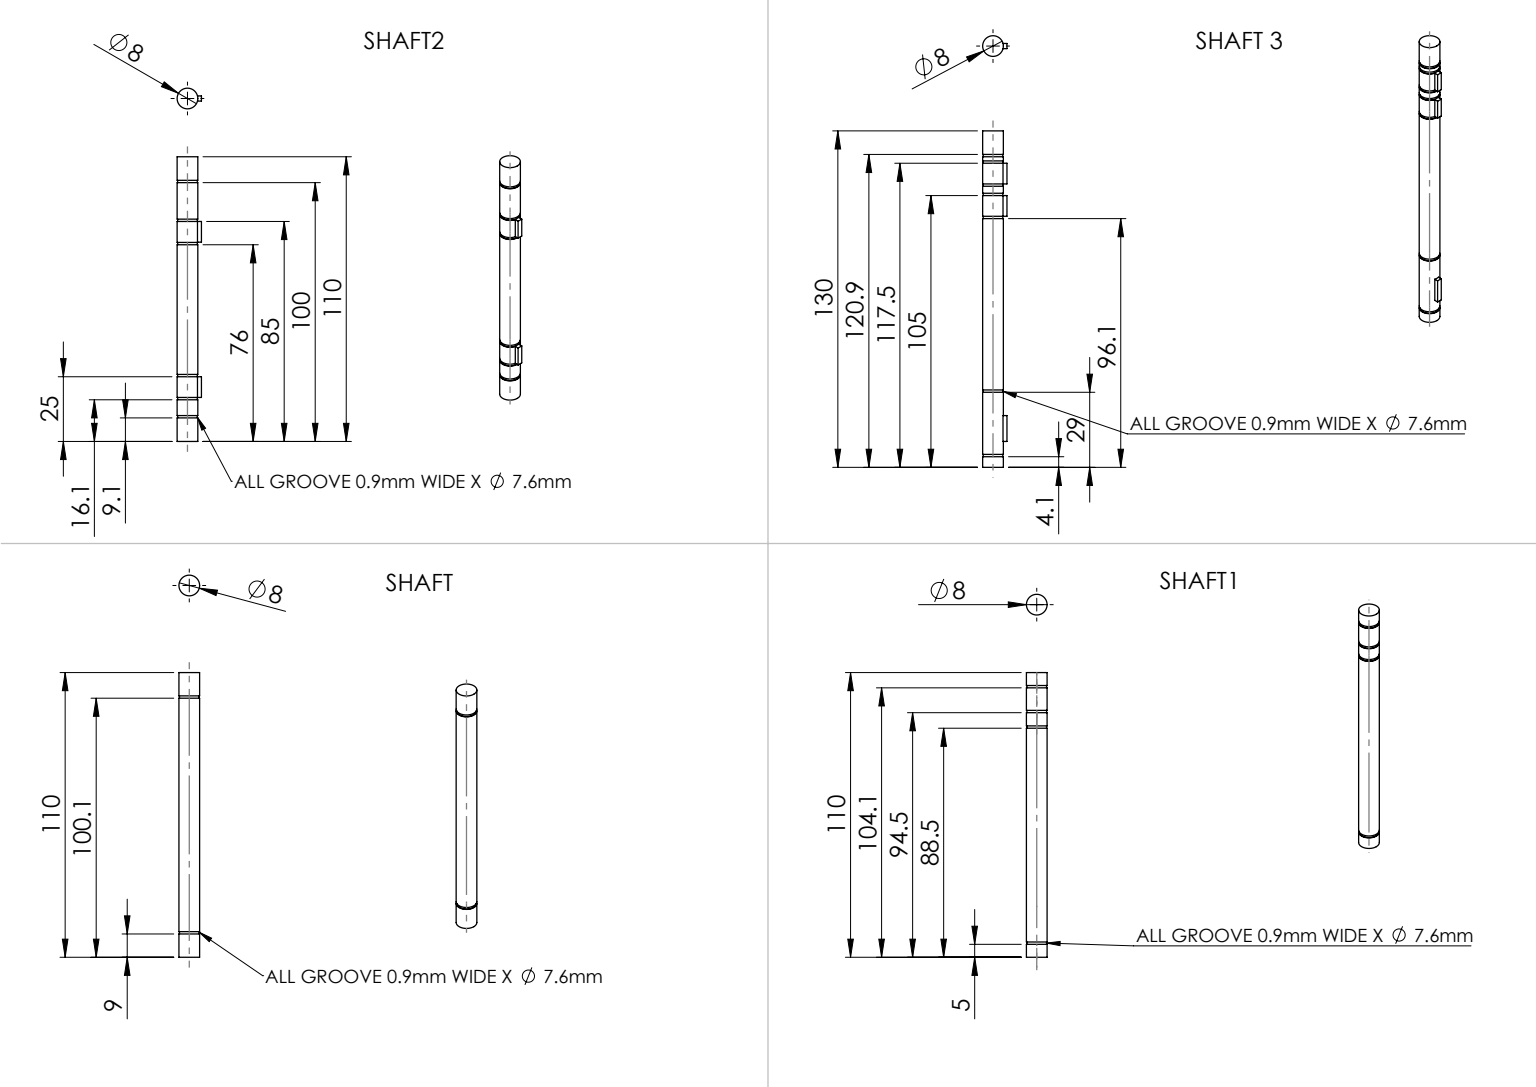
ISO-10303-21;
HEADER;
FILE_DESCRIPTION (('STEP AP214'),
    '1' );
FILE_NAME ('shaft.step',
    '2026-09-28T15:49:00',
    ( '' ),
    ( '' ),
    'SwSTEP 2.0',
    'SolidWorks 2026',
    '' );
FILE_SCHEMA (( 'AUTOMOTIVE_DESIGN' ));
ENDSEC;

DATA;
#80=ADVANCED_FACE ( 'NONE', ( #27547, #5915 ), #12161, .T. ) ;
#129=COLOUR_RGB ( '', 0.40784314, 0.44705882, 0.49803922) ;
#234=AXIS2_PLACEMENT_3D ( 'NONE', #3071, #14027, #25022 ) ;
#259=ADVANCED_FACE ( 'NONE', ( #12521 ), #20953, .T. ) ;
#263=CARTESIAN_POINT ( 'NONE',  ( 0.000000000000000000, -2.710505431213761085E-17, 54.99999999999999289 ) ) ;
#301=ORIENTED_EDGE ( 'NONE', *, *, #5401, .F. ) ;
#489=CARTESIAN_POINT ( 'NONE',  ( 4.000000000000000000, 4.627536653468036720E-16, 45.99999999999998579 ) ) ;
#517=DIRECTION ( 'NONE',  ( -1.000000000000000000, 0.000000000000000000, 0.000000000000000000 ) ) ;
#545=CIRCLE ( 'NONE', #10351, 4.000000000000000000 ) ;
#600=DIRECTION ( 'NONE',  ( -1.000000000000000000, 0.000000000000000000, 0.000000000000000000 ) ) ;
#613=FACE_OUTER_BOUND ( 'NONE', #17801, .T. ) ;
#665=PLANE ( 'NONE',  #1337 ) ;
#705=ADVANCED_FACE ( 'NONE', ( #23823 ), #18225, .T. ) ;
#706=DIRECTION ( 'NONE',  ( 1.000000000000000000, 0.000000000000000000, 0.000000000000000000 ) ) ;
#829=DIRECTION ( 'NONE',  ( 0.000000000000000000, 0.000000000000000000, -1.000000000000000000 ) ) ;
#842=VECTOR ( 'NONE', #18131, 1000.000000000000000 ) ;
#860=DIRECTION ( 'NONE',  ( 1.000000000000000000, 0.000000000000000000, 0.000000000000000000 ) ) ;
#903=CIRCLE ( 'NONE', #21584, 3.799999999999999822 ) ;
#937=SHAPE_REPRESENTATION_RELATIONSHIP ( 'NONE' , 'NONE' ,  #15534, #14621 ) ;
#1059=DIRECTION ( 'NONE',  ( 0.000000000000000000, 0.000000000000000000, -1.000000000000000000 ) ) ;
#1066=DIRECTION ( 'NONE',  ( 0.000000000000000000, 0.000000000000000000, -1.000000000000000000 ) ) ;
#1122=SURFACE_STYLE_USAGE ( .BOTH. , #3832 ) ;
#1124=EDGE_LOOP ( 'NONE', ( #30644, #31350 ) ) ;
#1169=EDGE_CURVE ( 'NONE', #3555, #2086, #8831, .T. ) ;
#1291=( LENGTH_UNIT ( ) NAMED_UNIT ( * ) SI_UNIT ( .MILLI., .METRE. ) );
#1322=CYLINDRICAL_SURFACE ( 'NONE', #32817, 3.799999999999999822 ) ;
#1337=AXIS2_PLACEMENT_3D ( 'NONE', #22806, #33808, #28399 ) ;
#1373=EDGE_LOOP ( 'NONE', ( #13603, #23594 ) ) ;
#1375=AXIS2_PLACEMENT_3D ( 'NONE', #34845, #33025, #24748 ) ;
#1477=DIRECTION ( 'NONE',  ( 0.000000000000000000, 0.000000000000000000, 1.000000000000000000 ) ) ;
#1539=DIRECTION ( 'NONE',  ( 0.000000000000000000, 0.000000000000000000, -1.000000000000000000 ) ) ;
#1577=AXIS2_PLACEMENT_3D ( 'NONE', #7509, #1763, #18490 ) ;
#1686=FACE_OUTER_BOUND ( 'NONE', #17486, .T. ) ;
#1753=EDGE_CURVE ( 'NONE', #16353, #3289, #16331, .T. ) ;
#1763=DIRECTION ( 'NONE',  ( 0.000000000000000000, 0.000000000000000000, -1.000000000000000000 ) ) ;
#1866=CARTESIAN_POINT ( 'NONE',  ( 0.000000000000000000, -2.710505431213761085E-17, 45.10000000000000142 ) ) ;
#1902=FACE_OUTER_BOUND ( 'NONE', #33338, .T. ) ;
#2086=VERTEX_POINT ( 'NONE', #489 ) ;
#2220=FACE_OUTER_BOUND ( 'NONE', #24548, .T. ) ;
#2301=AXIS2_PLACEMENT_3D ( 'NONE', #14881, #3933, #26600 ) ;
#2321=CARTESIAN_POINT ( 'NONE',  ( 0.000000000000000000, -2.710505431213761085E-17, -45.10000000000000142 ) ) ;
#2331=ADVANCED_FACE ( 'NONE', ( #31792 ), #18100, .T. ) ;
#2429=DIRECTION ( 'NONE',  ( 0.000000000000000000, 0.000000000000000000, -1.000000000000000000 ) ) ;
#2463=ORIENTED_EDGE ( 'NONE', *, *, #5481, .F. ) ;
#2522=APPLICATION_CONTEXT ( 'automotive_design' ) ;
#2817=AXIS2_PLACEMENT_3D ( 'NONE', #31798, #6779, #34335 ) ;
#2884=CARTESIAN_POINT ( 'NONE',  ( 0.000000000000000000, -2.710505431213761085E-17, -45.10000000000000142 ) ) ;
#2978=FILL_AREA_STYLE_COLOUR ( '', #129 ) ;
#3001=APPLICATION_CONTEXT ( 'automotive_design' ) ;
#3071=CARTESIAN_POINT ( 'NONE',  ( 0.000000000000000000, -2.710505431213761085E-17, -45.10000000000000142 ) ) ;
#3181=AXIS2_PLACEMENT_3D ( 'NONE', #2884, #32755, #11149 ) ;
#3219=CARTESIAN_POINT ( 'NONE',  ( 0.000000000000000000, -2.710505431213761085E-17, -54.99999999999999289 ) ) ;
#3289=VERTEX_POINT ( 'NONE', #18576 ) ;
#3320=DIRECTION ( 'NONE',  ( -1.000000000000000000, 0.000000000000000000, 0.000000000000000000 ) ) ;
#3382=CARTESIAN_POINT ( 'NONE',  ( 4.000000000000000000, 4.627536653468036720E-16, 45.10000000000000142 ) ) ;
#3555=VERTEX_POINT ( 'NONE', #12061 ) ;
#3639=AXIS2_PLACEMENT_3D ( 'NONE', #10281, #27025, #32239 ) ;
#3651=CARTESIAN_POINT ( 'NONE',  ( -3.799999999999999822, 4.382607293638566128E-16, 45.99999999999998579 ) ) ;
#3674=DIRECTION ( 'NONE',  ( 0.000000000000000000, 0.000000000000000000, -1.000000000000000000 ) ) ;
#3832=SURFACE_SIDE_STYLE ('',( #7220 ) ) ;
#3850=CARTESIAN_POINT ( 'NONE',  ( 0.000000000000000000, -2.710505431213761085E-17, 45.10000000000000142 ) ) ;
#3852=AXIS2_PLACEMENT_3D ( 'NONE', #24445, #10762, #21729 ) ;
#3933=DIRECTION ( 'NONE',  ( 0.000000000000000000, 0.000000000000000000, -1.000000000000000000 ) ) ;
#3969=CIRCLE ( 'NONE', #24668, 4.000000000000000000 ) ;
#4052=ORIENTED_EDGE ( 'NONE', *, *, #12390, .F. ) ;
#4364=FILL_AREA_STYLE_COLOUR ( '', #22512 ) ;
#4391=VECTOR ( 'NONE', #18228, 1000.000000000000000 ) ;
#4412=ORIENTED_EDGE ( 'NONE', *, *, #11688, .F. ) ;
#4594=AXIS2_PLACEMENT_3D ( 'NONE', #2321, #12751, #21197 ) ;
#4692=ADVANCED_FACE ( 'NONE', ( #1902 ), #12877, .T. ) ;
#4738=ORIENTED_EDGE ( 'NONE', *, *, #29385, .T. ) ;
#4795=LINE ( 'NONE', #15738, #14958 ) ;
#4961=AXIS2_PLACEMENT_3D ( 'NONE', #6185, #14096, #3320 ) ;
#4987=ORIENTED_EDGE ( 'NONE', *, *, #32459, .F. ) ;
#5002=AXIS2_PLACEMENT_3D ( 'NONE', #29082, #1539, #9453 ) ;
#5030=CIRCLE ( 'NONE', #26307, 3.799999999999999822 ) ;
#5259=ORIENTED_EDGE ( 'NONE', *, *, #9211, .F. ) ;
#5302=VECTOR ( 'NONE', #5780, 1000.000000000000000 ) ;
#5401=EDGE_CURVE ( 'NONE', #13238, #3289, #31820, .T. ) ;
#5481=EDGE_CURVE ( 'NONE', #19767, #30356, #11769, .T. ) ;
#5780=DIRECTION ( 'NONE',  ( 0.000000000000000000, 0.000000000000000000, -1.000000000000000000 ) ) ;
#5847=DIRECTION ( 'NONE',  ( -1.000000000000000000, 0.000000000000000000, 0.000000000000000000 ) ) ;
#5885=MECHANICAL_DESIGN_GEOMETRIC_PRESENTATION_REPRESENTATION('',(#8745),#32334);
#5915=FACE_OUTER_BOUND ( 'NONE', #1124, .T. ) ;
#6079=FACE_OUTER_BOUND ( 'NONE', #30683, .T. ) ;
#6185=CARTESIAN_POINT ( 'NONE',  ( 0.000000000000000000, -2.710505431213761085E-17, 45.10000000000000142 ) ) ;
#6239=EDGE_CURVE ( 'NONE', #13527, #8697, #34844, .T. ) ;
#6412=ORIENTED_EDGE ( 'NONE', *, *, #25778, .T. ) ;
#6415=CARTESIAN_POINT ( 'NONE',  ( 0.000000000000000000, -2.710505431213761085E-17, -45.10000000000000142 ) ) ;
#6460=CIRCLE ( 'NONE', #26601, 4.000000000000000000 ) ;
#6648=EDGE_CURVE ( 'NONE', #7361, #16353, #29410, .T. ) ;
#6779=DIRECTION ( 'NONE',  ( 0.000000000000000000, 0.000000000000000000, -1.000000000000000000 ) ) ;
#6807=CARTESIAN_POINT ( 'NONE',  ( 0.000000000000000000, -2.710505431213761085E-17, 45.99999999999998579 ) ) ;
#6995=MECHANICAL_DESIGN_GEOMETRIC_PRESENTATION_REPRESENTATION('',(#32297),#16755);
#7085=EDGE_CURVE ( 'NONE', #7361, #13238, #14160, .T. ) ;
#7154=CIRCLE ( 'NONE', #28440, 4.000000000000000000 ) ;
#7168=ORIENTED_EDGE ( 'NONE', *, *, #6239, .T. ) ;
#7220=SURFACE_STYLE_FILL_AREA ( #12453 ) ;
#7250=DIRECTION ( 'NONE',  ( 1.000000000000000000, 0.000000000000000000, 0.000000000000000000 ) ) ;
#7361=VERTEX_POINT ( 'NONE', #3382 ) ;
#7463=PRODUCT_DEFINITION_FORMATION_WITH_SPECIFIED_SOURCE ( 'ANY', '', #15545, .NOT_KNOWN. ) ;
#7509=CARTESIAN_POINT ( 'NONE',  ( 0.000000000000000000, -2.710505431213761085E-17, 45.99999999999998579 ) ) ;
#7548=DIRECTION ( 'NONE',  ( 0.000000000000000000, 0.000000000000000000, -1.000000000000000000 ) ) ;
#7803=AXIS2_PLACEMENT_3D ( 'NONE', #26250, #12925, #18316 ) ;
#7814=PRESENTATION_STYLE_ASSIGNMENT (( #10893 ) ) ;
#7886=CIRCLE ( 'NONE', #1577, 3.799999999999999822 ) ;
#7908=ORIENTED_EDGE ( 'NONE', *, *, #10208, .F. ) ;
#7979=ORIENTED_EDGE ( 'NONE', *, *, #9211, .T. ) ;
#8005=DIRECTION ( 'NONE',  ( 1.000000000000000000, 0.000000000000000000, 0.000000000000000000 ) ) ;
#8074=LINE ( 'NONE', #35463, #29789 ) ;
#8214=CARTESIAN_POINT ( 'NONE',  ( 0.000000000000000000, -2.710505431213761085E-17, 45.99999999999998579 ) ) ;
#8262=CARTESIAN_POINT ( 'NONE',  ( -3.799999999999999822, 4.382607293638566128E-16, 45.10000000000000142 ) ) ;
#8503=CARTESIAN_POINT ( 'NONE',  ( 0.000000000000000000, -2.710505431213761085E-17, 45.10000000000000142 ) ) ;
#8510=FACE_OUTER_BOUND ( 'NONE', #22264, .T. ) ;
#8538=DIRECTION ( 'NONE',  ( 0.000000000000000000, 0.000000000000000000, -1.000000000000000000 ) ) ;
#8581=ORIENTED_EDGE ( 'NONE', *, *, #5481, .T. ) ;
#8669=DIRECTION ( 'NONE',  ( -1.000000000000000000, 0.000000000000000000, 0.000000000000000000 ) ) ;
#8697=VERTEX_POINT ( 'NONE', #28414 ) ;
#8745=STYLED_ITEM ( 'NONE', ( #7814 ), #22652 ) ;
#8826=ORIENTED_EDGE ( 'NONE', *, *, #5401, .T. ) ;
#8827=PRODUCT_DEFINITION ( 'UNKNOWN', '', #7463, #25263 ) ;
#8831=LINE ( 'NONE', #23595, #14532 ) ;
#8949=LINE ( 'NONE', #17051, #16731 ) ;
#8986=ORIENTED_EDGE ( 'NONE', *, *, #10627, .F. ) ;
#9049=EDGE_CURVE ( 'NONE', #15222, #24982, #7886, .T. ) ;
#9170=EDGE_LOOP ( 'NONE', ( #9922, #6412, #7168, #12046 ) ) ;
#9211=EDGE_CURVE ( 'NONE', #24982, #15222, #5030, .T. ) ;
#9344=CIRCLE ( 'NONE', #17965, 3.799999999999999822 ) ;
#9453=DIRECTION ( 'NONE',  ( -1.000000000000000000, 0.000000000000000000, 0.000000000000000000 ) ) ;
#9506=CARTESIAN_POINT ( 'NONE',  ( -4.000000000000000000, -2.710505431213761085E-17, 54.99999999999999289 ) ) ;
#9622=ADVANCED_FACE ( 'NONE', ( #16968 ), #11414, .T. ) ;
#9922=ORIENTED_EDGE ( 'NONE', *, *, #12376, .T. ) ;
#10022=CIRCLE ( 'NONE', #14602, 3.799999999999999822 ) ;
#10134=DIRECTION ( 'NONE',  ( 0.000000000000000000, 0.000000000000000000, 1.000000000000000000 ) ) ;
#10208=EDGE_CURVE ( 'NONE', #3289, #16353, #24161, .T. ) ;
#10281=CARTESIAN_POINT ( 'NONE',  ( 0.000000000000000000, -2.710505431213761085E-17, 54.99999999999999289 ) ) ;
#10322=CARTESIAN_POINT ( 'NONE',  ( 0.000000000000000000, -2.710505431213761085E-17, 45.10000000000000142 ) ) ;
#10341=DIRECTION ( 'NONE',  ( 1.000000000000000000, 0.000000000000000000, 0.000000000000000000 ) ) ;
#10351=AXIS2_PLACEMENT_3D ( 'NONE', #3219, #14181, #19568 ) ;
#10491=ORIENTED_EDGE ( 'NONE', *, *, #25778, .F. ) ;
#10575=DIRECTION ( 'NONE',  ( 0.000000000000000000, 0.000000000000000000, -1.000000000000000000 ) ) ;
#10627=EDGE_CURVE ( 'NONE', #19767, #20378, #4795, .T. ) ;
#10693=DIRECTION ( 'NONE',  ( 0.000000000000000000, 0.000000000000000000, 1.000000000000000000 ) ) ;
#10762=DIRECTION ( 'NONE',  ( 0.000000000000000000, 0.000000000000000000, -1.000000000000000000 ) ) ;
#10825=CARTESIAN_POINT ( 'NONE',  ( 3.799999999999999822, -2.710505431213761085E-17, 45.10000000000000142 ) ) ;
#10893=SURFACE_STYLE_USAGE ( .BOTH. , #13583 ) ;
#11077=AXIS2_PLACEMENT_3D ( 'NONE', #16118, #32342, #27136 ) ;
#11099=ADVANCED_FACE ( 'NONE', ( #1686 ), #1322, .T. ) ;
#11149=DIRECTION ( 'NONE',  ( -1.000000000000000000, 0.000000000000000000, 0.000000000000000000 ) ) ;
#11171=CARTESIAN_POINT ( 'NONE',  ( 0.000000000000000000, -2.710505431213761085E-17, 54.99999999999999289 ) ) ;
#11189=ORIENTED_EDGE ( 'NONE', *, *, #25405, .F. ) ;
#11218=CARTESIAN_POINT ( 'NONE',  ( -3.799999999999999822, 4.382607293638566128E-16, 45.10000000000000142 ) ) ;
#11243=CARTESIAN_POINT ( 'NONE',  ( 0.000000000000000000, -2.710505431213761085E-17, -46.00000000000000000 ) ) ;
#11353=FACE_OUTER_BOUND ( 'NONE', #1373, .T. ) ;
#11414=CYLINDRICAL_SURFACE ( 'NONE', #29782, 4.000000000000000000 ) ;
#11521=PLANE ( 'NONE',  #18467 ) ;
#11646=FACE_BOUND ( 'NONE', #33527, .T. ) ;
#11688=EDGE_CURVE ( 'NONE', #30356, #28584, #8949, .T. ) ;
#11734=PLANE ( 'NONE',  #16422 ) ;
#11769=CIRCLE ( 'NONE', #12943, 3.799999999999999822 ) ;
#11877=ADVANCED_FACE ( 'NONE', ( #2220 ), #26871, .F. ) ;
#11899=VERTEX_POINT ( 'NONE', #13188 ) ;
#12029=CARTESIAN_POINT ( 'NONE',  ( 0.000000000000000000, -2.710505431213761085E-17, 54.99999999999999289 ) ) ;
#12030=DIRECTION ( 'NONE',  ( -1.000000000000000000, 0.000000000000000000, 0.000000000000000000 ) ) ;
#12046=ORIENTED_EDGE ( 'NONE', *, *, #18914, .F. ) ;
#12061=CARTESIAN_POINT ( 'NONE',  ( 4.000000000000000000, 4.627536653468036720E-16, 54.99999999999999289 ) ) ;
#12074=ORIENTED_EDGE ( 'NONE', *, *, #12143, .T. ) ;
#12094=PRESENTATION_STYLE_ASSIGNMENT (( #1122 ) ) ;
#12143=EDGE_CURVE ( 'NONE', #19005, #17954, #21792, .T. ) ;
#12161=PLANE ( 'NONE',  #3181 ) ;
#12211=DIRECTION ( 'NONE',  ( 0.000000000000000000, 0.000000000000000000, 1.000000000000000000 ) ) ;
#12292=DIRECTION ( 'NONE',  ( 0.000000000000000000, 0.000000000000000000, -1.000000000000000000 ) ) ;
#12358=CARTESIAN_POINT ( 'NONE',  ( 4.000000000000000000, 4.627536653468036720E-16, -46.00000000000000000 ) ) ;
#12376=EDGE_CURVE ( 'NONE', #11899, #35547, #28881, .T. ) ;
#12384=DIRECTION ( 'NONE',  ( 0.000000000000000000, 0.000000000000000000, -1.000000000000000000 ) ) ;
#12390=EDGE_CURVE ( 'NONE', #35547, #11899, #6460, .T. ) ;
#12453=FILL_AREA_STYLE ('',( #4364 ) ) ;
#12521=FACE_OUTER_BOUND ( 'NONE', #24417, .T. ) ;
#12557=ORIENTED_EDGE ( 'NONE', *, *, #32459, .T. ) ;
#12625=ORIENTED_EDGE ( 'NONE', *, *, #17612, .F. ) ;
#12725=DIRECTION ( 'NONE',  ( 0.000000000000000000, 0.000000000000000000, 1.000000000000000000 ) ) ;
#12751=DIRECTION ( 'NONE',  ( 0.000000000000000000, 0.000000000000000000, -1.000000000000000000 ) ) ;
#12877=CYLINDRICAL_SURFACE ( 'NONE', #1375, 4.000000000000000000 ) ;
#12925=DIRECTION ( 'NONE',  ( 0.000000000000000000, 0.000000000000000000, -1.000000000000000000 ) ) ;
#12943=AXIS2_PLACEMENT_3D ( 'NONE', #28601, #12384, #12030 ) ;
#13188=CARTESIAN_POINT ( 'NONE',  ( -4.000000000000000000, -2.710505431213761085E-17, -46.00000000000000000 ) ) ;
#13238=VERTEX_POINT ( 'NONE', #19194 ) ;
#13353=ORIENTED_EDGE ( 'NONE', *, *, #12376, .F. ) ;
#13527=VERTEX_POINT ( 'NONE', #32138 ) ;
#13583=SURFACE_SIDE_STYLE ('',( #35568 ) ) ;
#13603=ORIENTED_EDGE ( 'NONE', *, *, #16808, .T. ) ;
#13631=CARTESIAN_POINT ( 'NONE',  ( -3.799999999999999822, -2.710505431213761085E-17, -46.00000000000000000 ) ) ;
#13644=UNCERTAINTY_MEASURE_WITH_UNIT (LENGTH_MEASURE( 1.000000000000000082E-05 ), #23439, 'distance_accuracy_value', 'NONE');
#13913=FACE_BOUND ( 'NONE', #34994, .T. ) ;
#13947=FACE_OUTER_BOUND ( 'NONE', #31979, .T. ) ;
#14027=DIRECTION ( 'NONE',  ( 0.000000000000000000, 0.000000000000000000, -1.000000000000000000 ) ) ;
#14096=DIRECTION ( 'NONE',  ( 0.000000000000000000, 0.000000000000000000, -1.000000000000000000 ) ) ;
#14160=CIRCLE ( 'NONE', #3852, 4.000000000000000000 ) ;
#14163=ORIENTED_EDGE ( 'NONE', *, *, #25405, .T. ) ;
#14177=ORIENTED_EDGE ( 'NONE', *, *, #15082, .F. ) ;
#14181=DIRECTION ( 'NONE',  ( 0.000000000000000000, 0.000000000000000000, 1.000000000000000000 ) ) ;
#14198=LINE ( 'NONE', #8262, #17569 ) ;
#14203=VERTEX_POINT ( 'NONE', #15387 ) ;
#14428=DIRECTION ( 'NONE',  ( 0.000000000000000000, 0.000000000000000000, -1.000000000000000000 ) ) ;
#14459=DIRECTION ( 'NONE',  ( -1.000000000000000000, 0.000000000000000000, 0.000000000000000000 ) ) ;
#14492=ORIENTED_EDGE ( 'NONE', *, *, #10627, .T. ) ;
#14532=VECTOR ( 'NONE', #28823, 1000.000000000000000 ) ;
#14602=AXIS2_PLACEMENT_3D ( 'NONE', #28502, #12292, #31730 ) ;
#14621=ADVANCED_BREP_SHAPE_REPRESENTATION ( '', ( #22652, #21307 ), #24262 ) ;
#14690=CIRCLE ( 'NONE', #4961, 4.000000000000000000 ) ;
#14734=VECTOR ( 'NONE', #10575, 1000.000000000000000 ) ;
#14881=CARTESIAN_POINT ( 'NONE',  ( 0.000000000000000000, -2.710505431213761085E-17, 45.99999999999998579 ) ) ;
#14898=CIRCLE ( 'NONE', #2301, 4.000000000000000000 ) ;
#14913=ORIENTED_EDGE ( 'NONE', *, *, #6648, .T. ) ;
#14958=VECTOR ( 'NONE', #31961, 1000.000000000000000 ) ;
#15082=EDGE_CURVE ( 'NONE', #16940, #14203, #22822, .T. ) ;
#15210=ORIENTED_EDGE ( 'NONE', *, *, #12390, .T. ) ;
#15222=VERTEX_POINT ( 'NONE', #3651 ) ;
#15387=CARTESIAN_POINT ( 'NONE',  ( 3.799999999999999822, -2.710505431213761085E-17, 45.10000000000000142 ) ) ;
#15507=DIRECTION ( 'NONE',  ( -1.000000000000000000, 0.000000000000000000, 0.000000000000000000 ) ) ;
#15534=SHAPE_REPRESENTATION ( 'shaft', ( #21307 ), #24262 ) ;
#15545=PRODUCT ( 'shaft', 'shaft', '', ( #28755 ) ) ;
#15568=ORIENTED_EDGE ( 'NONE', *, *, #21852, .F. ) ;
#15715=ORIENTED_EDGE ( 'NONE', *, *, #7085, .F. ) ;
#15738=CARTESIAN_POINT ( 'NONE',  ( 3.799999999999999822, 4.382607293638566128E-16, -45.10000000000000142 ) ) ;
#16118=CARTESIAN_POINT ( 'NONE',  ( 0.000000000000000000, -2.710505431213761085E-17, -46.00000000000000000 ) ) ;
#16258=FILL_AREA_STYLE ('',( #2978 ) ) ;
#16263=CARTESIAN_POINT ( 'NONE',  ( 0.000000000000000000, -2.710505431213761085E-17, -54.99999999999999289 ) ) ;
#16331=CIRCLE ( 'NONE', #234, 4.000000000000000000 ) ;
#16353=VERTEX_POINT ( 'NONE', #25261 ) ;
#16379=CARTESIAN_POINT ( 'NONE',  ( -4.000000000000000000, -2.710505431213761085E-17, 54.99999999999999289 ) ) ;
#16408=DIRECTION ( 'NONE',  ( 0.000000000000000000, 0.000000000000000000, -1.000000000000000000 ) ) ;
#16422=AXIS2_PLACEMENT_3D ( 'NONE', #22706, #14428, #27620 ) ;
#16631=DIRECTION ( 'NONE',  ( 0.000000000000000000, 0.000000000000000000, 1.000000000000000000 ) ) ;
#16731=VECTOR ( 'NONE', #25717, 1000.000000000000000 ) ;
#16755=( GEOMETRIC_REPRESENTATION_CONTEXT ( 3 ) GLOBAL_UNCERTAINTY_ASSIGNED_CONTEXT ( ( #13644 ) ) GLOBAL_UNIT_ASSIGNED_CONTEXT ( ( #23439, #20712, #29015 ) ) REPRESENTATION_CONTEXT ( 'NONE', 'WORKASPACE' ) );
#16759=ORIENTED_EDGE ( 'NONE', *, *, #1169, .F. ) ;
#16808=EDGE_CURVE ( 'NONE', #19005, #3555, #3969, .T. ) ;
#16838=DIRECTION ( 'NONE',  ( 0.000000000000000000, 0.000000000000000000, -1.000000000000000000 ) ) ;
#16852=UNCERTAINTY_MEASURE_WITH_UNIT (LENGTH_MEASURE( 1.000000000000000082E-05 ), #1291, 'distance_accuracy_value', 'NONE');
#16920=AXIS2_PLACEMENT_3D ( 'NONE', #6415, #829, #29102 ) ;
#16940=VERTEX_POINT ( 'NONE', #11218 ) ;
#16968=FACE_OUTER_BOUND ( 'NONE', #30734, .T. ) ;
#17051=CARTESIAN_POINT ( 'NONE',  ( -3.799999999999999822, -2.710505431213761085E-17, -45.10000000000000142 ) ) ;
#17062=CARTESIAN_POINT ( 'NONE',  ( 0.000000000000000000, -2.710505431213761085E-17, 54.99999999999999289 ) ) ;
#17486=EDGE_LOOP ( 'NONE', ( #14177, #24005, #19107, #22794 ) ) ;
#17569=VECTOR ( 'NONE', #33120, 1000.000000000000000 ) ;
#17612=EDGE_CURVE ( 'NONE', #8697, #13527, #545, .T. ) ;
#17801=EDGE_LOOP ( 'NONE', ( #16759, #19908, #12074, #30354 ) ) ;
#17954=VERTEX_POINT ( 'NONE', #29653 ) ;
#17965=AXIS2_PLACEMENT_3D ( 'NONE', #22666, #2429, #21842 ) ;
#17971=ORIENTED_EDGE ( 'NONE', *, *, #15082, .T. ) ;
#18100=CYLINDRICAL_SURFACE ( 'NONE', #16920, 3.799999999999999822 ) ;
#18131=DIRECTION ( 'NONE',  ( 0.000000000000000000, 0.000000000000000000, -1.000000000000000000 ) ) ;
#18225=CYLINDRICAL_SURFACE ( 'NONE', #25462, 3.799999999999999822 ) ;
#18228=DIRECTION ( 'NONE',  ( 0.000000000000000000, 0.000000000000000000, -1.000000000000000000 ) ) ;
#18292=DIRECTION ( 'NONE',  ( 1.000000000000000000, 0.000000000000000000, 0.000000000000000000 ) ) ;
#18316=DIRECTION ( 'NONE',  ( -1.000000000000000000, 0.000000000000000000, 0.000000000000000000 ) ) ;
#18440=PRODUCT_DEFINITION_SHAPE ( 'NONE', 'NONE',  #8827 ) ;
#18467=AXIS2_PLACEMENT_3D ( 'NONE', #11171, #19951, #706 ) ;
#18490=DIRECTION ( 'NONE',  ( -1.000000000000000000, 0.000000000000000000, 0.000000000000000000 ) ) ;
#18576=CARTESIAN_POINT ( 'NONE',  ( -4.000000000000000000, -2.710505431213761085E-17, -45.10000000000000142 ) ) ;
#18914=EDGE_CURVE ( 'NONE', #11899, #8697, #8074, .T. ) ;
#19005=VERTEX_POINT ( 'NONE', #29470 ) ;
#19041=ADVANCED_FACE ( 'NONE', ( #34877 ), #26593, .T. ) ;
#19107=ORIENTED_EDGE ( 'NONE', *, *, #9049, .T. ) ;
#19128=CARTESIAN_POINT ( 'NONE',  ( -3.799999999999999822, -2.710505431213761085E-17, -45.10000000000000142 ) ) ;
#19194=CARTESIAN_POINT ( 'NONE',  ( -4.000000000000000000, -2.710505431213761085E-17, 45.10000000000000142 ) ) ;
#19323=( NAMED_UNIT ( * ) SI_UNIT ( $, .STERADIAN. ) SOLID_ANGLE_UNIT ( ) );
#19393=ORIENTED_EDGE ( 'NONE', *, *, #12143, .F. ) ;
#19514=DIRECTION ( 'NONE',  ( 0.000000000000000000, 0.000000000000000000, -1.000000000000000000 ) ) ;
#19558=EDGE_CURVE ( 'NONE', #2086, #17954, #14898, .T. ) ;
#19568=DIRECTION ( 'NONE',  ( 1.000000000000000000, 0.000000000000000000, 0.000000000000000000 ) ) ;
#19767=VERTEX_POINT ( 'NONE', #29652 ) ;
#19844=AXIS2_PLACEMENT_3D ( 'NONE', #16263, #16631, #8005 ) ;
#19908=ORIENTED_EDGE ( 'NONE', *, *, #16808, .F. ) ;
#19911=ORIENTED_EDGE ( 'NONE', *, *, #24261, .F. ) ;
#19951=DIRECTION ( 'NONE',  ( 0.000000000000000000, 0.000000000000000000, 1.000000000000000000 ) ) ;
#20293=DIRECTION ( 'NONE',  ( -1.000000000000000000, 0.000000000000000000, 0.000000000000000000 ) ) ;
#20378=VERTEX_POINT ( 'NONE', #22368 ) ;
#20712=( NAMED_UNIT ( * ) PLANE_ANGLE_UNIT ( ) SI_UNIT ( $, .RADIAN. ) );
#20782=AXIS2_PLACEMENT_3D ( 'NONE', #34613, #1477, #29022 ) ;
#20953=CYLINDRICAL_SURFACE ( 'NONE', #5002, 3.799999999999999822 ) ;
#21026=CIRCLE ( 'NONE', #35423, 4.000000000000000000 ) ;
#21197=DIRECTION ( 'NONE',  ( -1.000000000000000000, 0.000000000000000000, 0.000000000000000000 ) ) ;
#21307=AXIS2_PLACEMENT_3D ( 'NONE', #26589, #12725, #18292 ) ;
#21418=FACE_OUTER_BOUND ( 'NONE', #32308, .T. ) ;
#21474=CARTESIAN_POINT ( 'NONE',  ( 0.000000000000000000, -2.710505431213761085E-17, 54.99999999999999289 ) ) ;
#21584=AXIS2_PLACEMENT_3D ( 'NONE', #3850, #31729, #15507 ) ;
#21585=CYLINDRICAL_SURFACE ( 'NONE', #3639, 4.000000000000000000 ) ;
#21599=EDGE_CURVE ( 'NONE', #13238, #7361, #14690, .T. ) ;
#21729=DIRECTION ( 'NONE',  ( -1.000000000000000000, 0.000000000000000000, 0.000000000000000000 ) ) ;
#21792=LINE ( 'NONE', #16379, #5302 ) ;
#21842=DIRECTION ( 'NONE',  ( -1.000000000000000000, 0.000000000000000000, 0.000000000000000000 ) ) ;
#21852=EDGE_CURVE ( 'NONE', #14203, #16940, #903, .T. ) ;
#22075=DIRECTION ( 'NONE',  ( -1.000000000000000000, 0.000000000000000000, 0.000000000000000000 ) ) ;
#22218=ORIENTED_EDGE ( 'NONE', *, *, #9049, .F. ) ;
#22264=EDGE_LOOP ( 'NONE', ( #31167, #15715 ) ) ;
#22368=CARTESIAN_POINT ( 'NONE',  ( 3.799999999999999822, 4.382607293638566128E-16, -46.00000000000000000 ) ) ;
#22512=COLOUR_RGB ( '', 0.40784314, 0.44705882, 0.49803922) ;
#22652=MANIFOLD_SOLID_BREP ( 'Mirror1', #29050 ) ;
#22666=CARTESIAN_POINT ( 'NONE',  ( 0.000000000000000000, -2.710505431213761085E-17, -46.00000000000000000 ) ) ;
#22706=CARTESIAN_POINT ( 'NONE',  ( 0.000000000000000000, -2.710505431213761085E-17, 45.10000000000000142 ) ) ;
#22794=ORIENTED_EDGE ( 'NONE', *, *, #29385, .F. ) ;
#22806=CARTESIAN_POINT ( 'NONE',  ( 0.000000000000000000, -2.710505431213761085E-17, 45.99999999999998579 ) ) ;
#22822=CIRCLE ( 'NONE', #35503, 3.799999999999999822 ) ;
#22924=ORIENTED_EDGE ( 'NONE', *, *, #17612, .T. ) ;
#23248=( NAMED_UNIT ( * ) SI_UNIT ( $, .STERADIAN. ) SOLID_ANGLE_UNIT ( ) );
#23439=( LENGTH_UNIT ( ) NAMED_UNIT ( * ) SI_UNIT ( .MILLI., .METRE. ) );
#23594=ORIENTED_EDGE ( 'NONE', *, *, #25273, .T. ) ;
#23595=CARTESIAN_POINT ( 'NONE',  ( 4.000000000000000000, 4.627536653468036720E-16, 54.99999999999999289 ) ) ;
#23620=( NAMED_UNIT ( * ) PLANE_ANGLE_UNIT ( ) SI_UNIT ( $, .RADIAN. ) );
#23646=EDGE_LOOP ( 'NONE', ( #32024, #14913, #7908, #301 ) ) ;
#23727=ADVANCED_FACE ( 'NONE', ( #6079, #11646 ), #665, .T. ) ;
#23793=LINE ( 'NONE', #10825, #26318 ) ;
#23823=FACE_OUTER_BOUND ( 'NONE', #34061, .T. ) ;
#23934=AXIS2_PLACEMENT_3D ( 'NONE', #17062, #1059, #517 ) ;
#24005=ORIENTED_EDGE ( 'NONE', *, *, #28040, .T. ) ;
#24161=CIRCLE ( 'NONE', #4594, 4.000000000000000000 ) ;
#24252=CARTESIAN_POINT ( 'NONE',  ( 0.000000000000000000, -2.710505431213761085E-17, -46.00000000000000000 ) ) ;
#24261=EDGE_CURVE ( 'NONE', #30356, #19767, #10022, .T. ) ;
#24262=( GEOMETRIC_REPRESENTATION_CONTEXT ( 3 ) GLOBAL_UNCERTAINTY_ASSIGNED_CONTEXT ( ( #16852 ) ) GLOBAL_UNIT_ASSIGNED_CONTEXT ( ( #1291, #23620, #23248 ) ) REPRESENTATION_CONTEXT ( 'NONE', 'WORKASPACE' ) );
#24267=LINE ( 'NONE', #35254, #14734 ) ;
#24417=EDGE_LOOP ( 'NONE', ( #30820, #14492, #4987, #4412 ) ) ;
#24445=CARTESIAN_POINT ( 'NONE',  ( 0.000000000000000000, -2.710505431213761085E-17, 45.10000000000000142 ) ) ;
#24548=EDGE_LOOP ( 'NONE', ( #12625, #35137 ) ) ;
#24668=AXIS2_PLACEMENT_3D ( 'NONE', #21474, #10693, #10341 ) ;
#24748=DIRECTION ( 'NONE',  ( -1.000000000000000000, 0.000000000000000000, 0.000000000000000000 ) ) ;
#24852=ORIENTED_EDGE ( 'NONE', *, *, #18914, .T. ) ;
#24935=PLANE ( 'NONE',  #27924 ) ;
#24982=VERTEX_POINT ( 'NONE', #29710 ) ;
#25022=DIRECTION ( 'NONE',  ( -1.000000000000000000, 0.000000000000000000, 0.000000000000000000 ) ) ;
#25113=CYLINDRICAL_SURFACE ( 'NONE', #30337, 4.000000000000000000 ) ;
#25261=CARTESIAN_POINT ( 'NONE',  ( 4.000000000000000000, 4.627536653468036720E-16, -45.10000000000000142 ) ) ;
#25263=PRODUCT_DEFINITION_CONTEXT ( 'detailed design', #3001, 'design' ) ;
#25273=EDGE_CURVE ( 'NONE', #3555, #19005, #21026, .T. ) ;
#25335=ADVANCED_FACE ( 'NONE', ( #30938 ), #28600, .T. ) ;
#25405=EDGE_CURVE ( 'NONE', #20378, #28584, #27932, .T. ) ;
#25462=AXIS2_PLACEMENT_3D ( 'NONE', #1866, #34807, #34266 ) ;
#25574=ORIENTED_EDGE ( 'NONE', *, *, #25273, .F. ) ;
#25717=DIRECTION ( 'NONE',  ( 0.000000000000000000, 0.000000000000000000, -1.000000000000000000 ) ) ;
#25778=EDGE_CURVE ( 'NONE', #35547, #13527, #24267, .T. ) ;
#26250=CARTESIAN_POINT ( 'NONE',  ( 0.000000000000000000, -2.710505431213761085E-17, -46.00000000000000000 ) ) ;
#26307=AXIS2_PLACEMENT_3D ( 'NONE', #8214, #16838, #22075 ) ;
#26318=VECTOR ( 'NONE', #34776, 1000.000000000000000 ) ;
#26481=ADVANCED_FACE ( 'NONE', ( #21418 ), #21585, .T. ) ;
#26589=CARTESIAN_POINT ( 'NONE',  ( 0.000000000000000000, 0.000000000000000000, 0.000000000000000000 ) ) ;
#26593=CYLINDRICAL_SURFACE ( 'NONE', #2817, 4.000000000000000000 ) ;
#26600=DIRECTION ( 'NONE',  ( -1.000000000000000000, 0.000000000000000000, 0.000000000000000000 ) ) ;
#26601=AXIS2_PLACEMENT_3D ( 'NONE', #24252, #35239, #30012 ) ;
#26861=EDGE_CURVE ( 'NONE', #17954, #2086, #7154, .T. ) ;
#26871=PLANE ( 'NONE',  #20782 ) ;
#26933=( NAMED_UNIT ( * ) PLANE_ANGLE_UNIT ( ) SI_UNIT ( $, .RADIAN. ) );
#27025=DIRECTION ( 'NONE',  ( 0.000000000000000000, 0.000000000000000000, -1.000000000000000000 ) ) ;
#27102=( LENGTH_UNIT ( ) NAMED_UNIT ( * ) SI_UNIT ( .MILLI., .METRE. ) );
#27136=DIRECTION ( 'NONE',  ( -1.000000000000000000, 0.000000000000000000, 0.000000000000000000 ) ) ;
#27547=FACE_BOUND ( 'NONE', #31844, .T. ) ;
#27559=ORIENTED_EDGE ( 'NONE', *, *, #21852, .T. ) ;
#27620=DIRECTION ( 'NONE',  ( -1.000000000000000000, 0.000000000000000000, 0.000000000000000000 ) ) ;
#27722=ADVANCED_FACE ( 'NONE', ( #33038, #13947 ), #24935, .F. ) ;
#27924=AXIS2_PLACEMENT_3D ( 'NONE', #11243, #8538, #5847 ) ;
#27932=CIRCLE ( 'NONE', #7803, 3.799999999999999822 ) ;
#28040=EDGE_CURVE ( 'NONE', #16940, #15222, #14198, .T. ) ;
#28055=ORIENTED_EDGE ( 'NONE', *, *, #11688, .T. ) ;
#28327=CARTESIAN_POINT ( 'NONE',  ( 0.000000000000000000, -2.710505431213761085E-17, 54.99999999999999289 ) ) ;
#28399=DIRECTION ( 'NONE',  ( -1.000000000000000000, 0.000000000000000000, 0.000000000000000000 ) ) ;
#28414=CARTESIAN_POINT ( 'NONE',  ( -4.000000000000000000, -2.710505431213761085E-17, -54.99999999999999289 ) ) ;
#28440=AXIS2_PLACEMENT_3D ( 'NONE', #6807, #1066, #20293 ) ;
#28502=CARTESIAN_POINT ( 'NONE',  ( 0.000000000000000000, -2.710505431213761085E-17, -45.10000000000000142 ) ) ;
#28584=VERTEX_POINT ( 'NONE', #13631 ) ;
#28600=CYLINDRICAL_SURFACE ( 'NONE', #23934, 4.000000000000000000 ) ;
#28601=CARTESIAN_POINT ( 'NONE',  ( 0.000000000000000000, -2.710505431213761085E-17, -45.10000000000000142 ) ) ;
#28755=PRODUCT_CONTEXT ( 'NONE', #2522, 'mechanical' ) ;
#28823=DIRECTION ( 'NONE',  ( 0.000000000000000000, 0.000000000000000000, -1.000000000000000000 ) ) ;
#28881=CIRCLE ( 'NONE', #11077, 4.000000000000000000 ) ;
#29015=( NAMED_UNIT ( * ) SI_UNIT ( $, .STERADIAN. ) SOLID_ANGLE_UNIT ( ) );
#29022=DIRECTION ( 'NONE',  ( 1.000000000000000000, 0.000000000000000000, 0.000000000000000000 ) ) ;
#29050=CLOSED_SHELL ( 'NONE', ( #4692, #11099, #19041, #259, #25335, #9622, #80, #27722, #2331, #11877, #26481, #30453, #23727, #705, #31075, #33316 ) ) ;
#29057=ORIENTED_EDGE ( 'NONE', *, *, #28040, .F. ) ;
#29082=CARTESIAN_POINT ( 'NONE',  ( 0.000000000000000000, -2.710505431213761085E-17, -45.10000000000000142 ) ) ;
#29102=DIRECTION ( 'NONE',  ( -1.000000000000000000, 0.000000000000000000, 0.000000000000000000 ) ) ;
#29385=EDGE_CURVE ( 'NONE', #14203, #24982, #23793, .T. ) ;
#29410=LINE ( 'NONE', #31913, #4391 ) ;
#29470=CARTESIAN_POINT ( 'NONE',  ( -4.000000000000000000, -2.710505431213761085E-17, 54.99999999999999289 ) ) ;
#29652=CARTESIAN_POINT ( 'NONE',  ( 3.799999999999999822, 4.382607293638566128E-16, -45.10000000000000142 ) ) ;
#29653=CARTESIAN_POINT ( 'NONE',  ( -4.000000000000000000, -2.710505431213761085E-17, 45.99999999999998579 ) ) ;
#29688=EDGE_LOOP ( 'NONE', ( #8986, #8581, #28055, #11189 ) ) ;
#29710=CARTESIAN_POINT ( 'NONE',  ( 3.799999999999999822, -2.710505431213761085E-17, 45.99999999999998579 ) ) ;
#29765=ORIENTED_EDGE ( 'NONE', *, *, #1753, .F. ) ;
#29782=AXIS2_PLACEMENT_3D ( 'NONE', #28327, #3674, #600 ) ;
#29789=VECTOR ( 'NONE', #7548, 1000.000000000000000 ) ;
#30012=DIRECTION ( 'NONE',  ( -1.000000000000000000, 0.000000000000000000, 0.000000000000000000 ) ) ;
#30337=AXIS2_PLACEMENT_3D ( 'NONE', #263, #19514, #14459 ) ;
#30354=ORIENTED_EDGE ( 'NONE', *, *, #19558, .F. ) ;
#30356=VERTEX_POINT ( 'NONE', #19128 ) ;
#30453=ADVANCED_FACE ( 'NONE', ( #8510, #13913 ), #11734, .F. ) ;
#30644=ORIENTED_EDGE ( 'NONE', *, *, #10208, .T. ) ;
#30683=EDGE_LOOP ( 'NONE', ( #31165, #34687 ) ) ;
#30734=EDGE_LOOP ( 'NONE', ( #32367, #31323, #8826, #29765 ) ) ;
#30745=ORIENTED_EDGE ( 'NONE', *, *, #26861, .F. ) ;
#30820=ORIENTED_EDGE ( 'NONE', *, *, #24261, .T. ) ;
#30938=FACE_OUTER_BOUND ( 'NONE', #23646, .T. ) ;
#31075=ADVANCED_FACE ( 'NONE', ( #11353 ), #11521, .T. ) ;
#31165=ORIENTED_EDGE ( 'NONE', *, *, #26861, .T. ) ;
#31167=ORIENTED_EDGE ( 'NONE', *, *, #21599, .F. ) ;
#31323=ORIENTED_EDGE ( 'NONE', *, *, #7085, .T. ) ;
#31350=ORIENTED_EDGE ( 'NONE', *, *, #1753, .T. ) ;
#31593=UNCERTAINTY_MEASURE_WITH_UNIT (LENGTH_MEASURE( 1.000000000000000082E-05 ), #27102, 'distance_accuracy_value', 'NONE');
#31729=DIRECTION ( 'NONE',  ( 0.000000000000000000, 0.000000000000000000, -1.000000000000000000 ) ) ;
#31730=DIRECTION ( 'NONE',  ( -1.000000000000000000, 0.000000000000000000, 0.000000000000000000 ) ) ;
#31792=FACE_OUTER_BOUND ( 'NONE', #29688, .T. ) ;
#31798=CARTESIAN_POINT ( 'NONE',  ( 0.000000000000000000, -2.710505431213761085E-17, 54.99999999999999289 ) ) ;
#31820=LINE ( 'NONE', #9506, #842 ) ;
#31844=EDGE_LOOP ( 'NONE', ( #19911, #2463 ) ) ;
#31913=CARTESIAN_POINT ( 'NONE',  ( 4.000000000000000000, 4.627536653468036720E-16, 54.99999999999999289 ) ) ;
#31961=DIRECTION ( 'NONE',  ( 0.000000000000000000, 0.000000000000000000, -1.000000000000000000 ) ) ;
#31979=EDGE_LOOP ( 'NONE', ( #13353, #4052 ) ) ;
#32024=ORIENTED_EDGE ( 'NONE', *, *, #21599, .T. ) ;
#32138=CARTESIAN_POINT ( 'NONE',  ( 4.000000000000000000, 4.627536653468036720E-16, -54.99999999999999289 ) ) ;
#32239=DIRECTION ( 'NONE',  ( -1.000000000000000000, 0.000000000000000000, 0.000000000000000000 ) ) ;
#32297=STYLED_ITEM ( 'NONE', ( #12094 ), #14621 ) ;
#32308=EDGE_LOOP ( 'NONE', ( #10491, #15210, #24852, #22924 ) ) ;
#32334=( GEOMETRIC_REPRESENTATION_CONTEXT ( 3 ) GLOBAL_UNCERTAINTY_ASSIGNED_CONTEXT ( ( #31593 ) ) GLOBAL_UNIT_ASSIGNED_CONTEXT ( ( #27102, #26933, #19323 ) ) REPRESENTATION_CONTEXT ( 'NONE', 'WORKASPACE' ) );
#32342=DIRECTION ( 'NONE',  ( 0.000000000000000000, 0.000000000000000000, -1.000000000000000000 ) ) ;
#32367=ORIENTED_EDGE ( 'NONE', *, *, #6648, .F. ) ;
#32459=EDGE_CURVE ( 'NONE', #28584, #20378, #9344, .T. ) ;
#32755=DIRECTION ( 'NONE',  ( 0.000000000000000000, 0.000000000000000000, -1.000000000000000000 ) ) ;
#32817=AXIS2_PLACEMENT_3D ( 'NONE', #10322, #10134, #7250 ) ;
#33025=DIRECTION ( 'NONE',  ( 0.000000000000000000, 0.000000000000000000, -1.000000000000000000 ) ) ;
#33038=FACE_BOUND ( 'NONE', #33290, .T. ) ;
#33120=DIRECTION ( 'NONE',  ( 0.000000000000000000, 0.000000000000000000, 1.000000000000000000 ) ) ;
#33290=EDGE_LOOP ( 'NONE', ( #12557, #14163 ) ) ;
#33316=ADVANCED_FACE ( 'NONE', ( #613 ), #25113, .T. ) ;
#33338=EDGE_LOOP ( 'NONE', ( #25574, #34090, #30745, #19393 ) ) ;
#33527=EDGE_LOOP ( 'NONE', ( #5259, #22218 ) ) ;
#33808=DIRECTION ( 'NONE',  ( 0.000000000000000000, 0.000000000000000000, -1.000000000000000000 ) ) ;
#34061=EDGE_LOOP ( 'NONE', ( #29057, #15568, #4738, #7979 ) ) ;
#34090=ORIENTED_EDGE ( 'NONE', *, *, #1169, .T. ) ;
#34158=SHAPE_DEFINITION_REPRESENTATION ( #18440, #15534 ) ;
#34266=DIRECTION ( 'NONE',  ( 1.000000000000000000, 0.000000000000000000, 0.000000000000000000 ) ) ;
#34335=DIRECTION ( 'NONE',  ( -1.000000000000000000, 0.000000000000000000, 0.000000000000000000 ) ) ;
#34613=CARTESIAN_POINT ( 'NONE',  ( 0.000000000000000000, -2.710505431213761085E-17, -54.99999999999999289 ) ) ;
#34687=ORIENTED_EDGE ( 'NONE', *, *, #19558, .T. ) ;
#34776=DIRECTION ( 'NONE',  ( 0.000000000000000000, 0.000000000000000000, 1.000000000000000000 ) ) ;
#34807=DIRECTION ( 'NONE',  ( 0.000000000000000000, 0.000000000000000000, 1.000000000000000000 ) ) ;
#34844=CIRCLE ( 'NONE', #19844, 4.000000000000000000 ) ;
#34845=CARTESIAN_POINT ( 'NONE',  ( 0.000000000000000000, -2.710505431213761085E-17, 54.99999999999999289 ) ) ;
#34877=FACE_OUTER_BOUND ( 'NONE', #9170, .T. ) ;
#34994=EDGE_LOOP ( 'NONE', ( #27559, #17971 ) ) ;
#35137=ORIENTED_EDGE ( 'NONE', *, *, #6239, .F. ) ;
#35239=DIRECTION ( 'NONE',  ( 0.000000000000000000, 0.000000000000000000, -1.000000000000000000 ) ) ;
#35254=CARTESIAN_POINT ( 'NONE',  ( 4.000000000000000000, 4.627536653468036720E-16, 54.99999999999999289 ) ) ;
#35423=AXIS2_PLACEMENT_3D ( 'NONE', #12029, #12211, #860 ) ;
#35463=CARTESIAN_POINT ( 'NONE',  ( -4.000000000000000000, -2.710505431213761085E-17, 54.99999999999999289 ) ) ;
#35503=AXIS2_PLACEMENT_3D ( 'NONE', #8503, #16408, #8669 ) ;
#35547=VERTEX_POINT ( 'NONE', #12358 ) ;
#35568=SURFACE_STYLE_FILL_AREA ( #16258 ) ;
ENDSEC;
END-ISO-10303-21;
